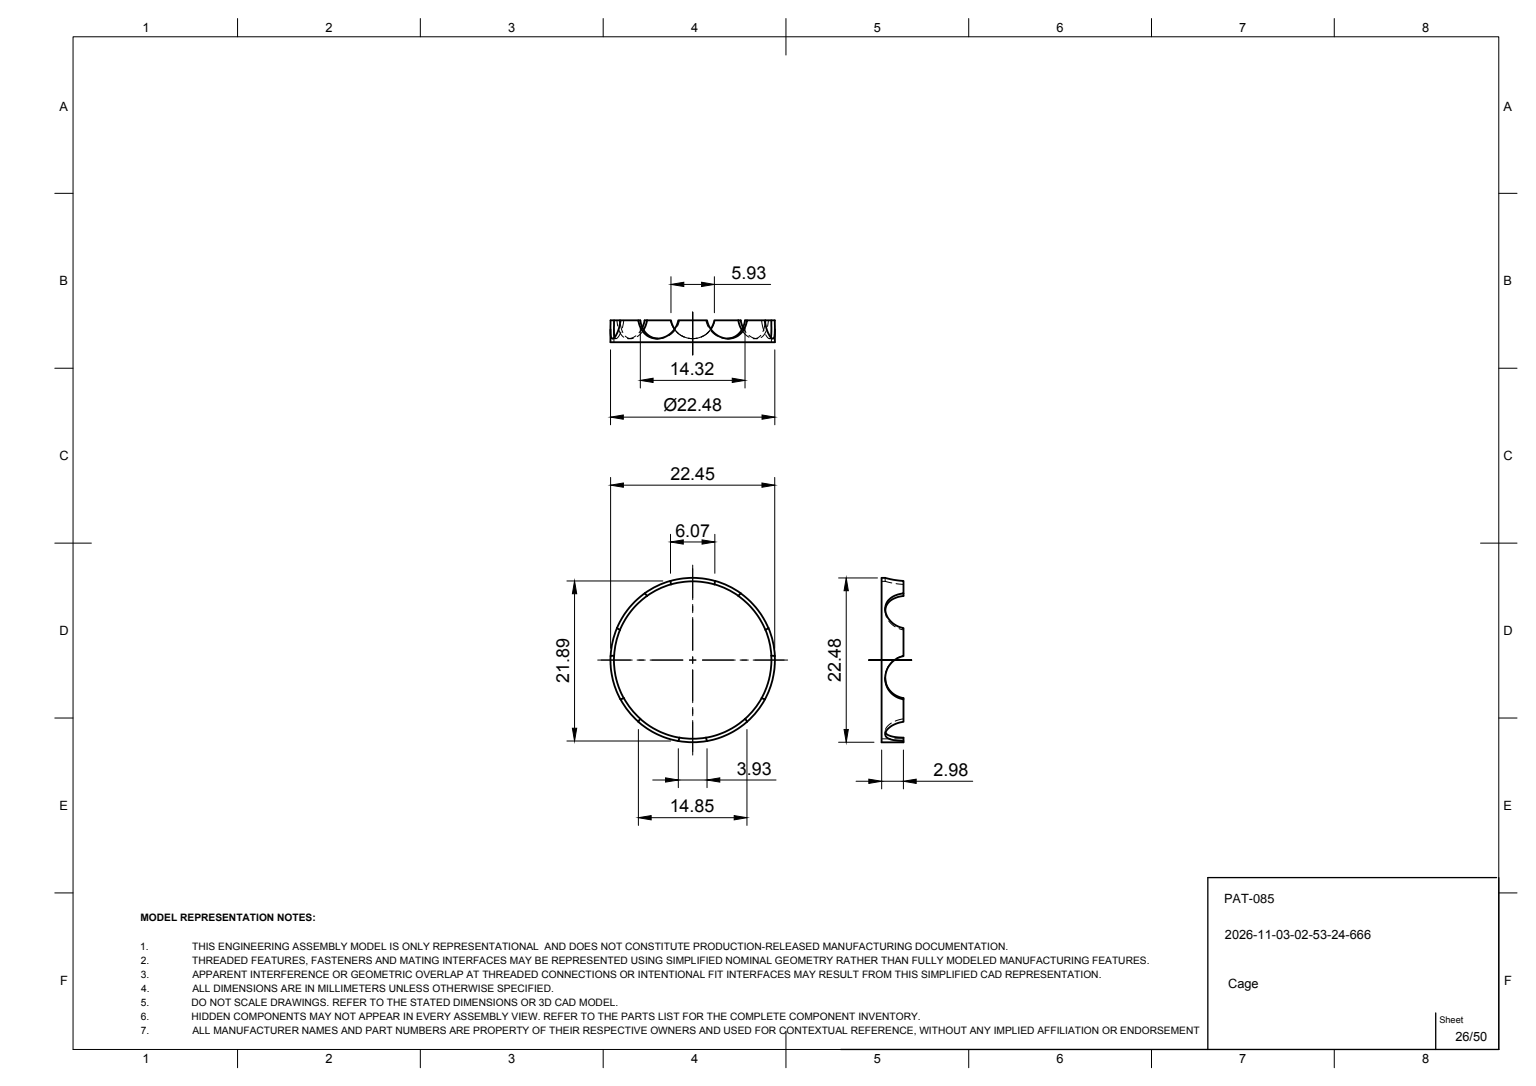
ISO-10303-21;
HEADER;
/* Generated by software containing ST-Developer
 * from STEP Tools, Inc. (www.steptools.com) 
 */

FILE_DESCRIPTION(
/* description */ ('Rack and pinion manual slide'),
/* implementation_level */ '2;1');

FILE_NAME(
/* name */ 'Cage.step',
/* time_stamp */ '2026-10-28T03:22:49-07:00',
/* author */ (''),
/* organization */ (''),
/* preprocessor_version */ 'ST-DEVELOPER v20.2',
/* originating_system */ 'Autodesk Translation Framework v15.17.0.0',
/* authorisation */ '');

FILE_SCHEMA (('AUTOMOTIVE_DESIGN { 1 0 10303 214 3 1 1 }'));
ENDSEC;

DATA;
#10=MECHANICAL_DESIGN_GEOMETRIC_PRESENTATION_REPRESENTATION('',(#760),#34851);
#575=B_SPLINE_CURVE_WITH_KNOTS('',3,(#20890,#20891,#20892,#20893,#20894,
#20895,#20896,#20897,#20898,#20899,#20900,#20901,#20902,#20903,#20904,#20905,
#20906,#20907,#20908,#20909,#20910,#20911),.UNSPECIFIED.,.F.,.F.,(4,2,2,
2,2,2,2,2,2,2,4),(0.0591825211272536,0.157966726598481,0.236950089897721,
0.315933453196962,0.391576304923761,0.46721915665056,0.54286200837736,0.618504860104159,
0.697488223403399,0.77647158670264,0.875255792173867),.UNSPECIFIED.);
#576=B_SPLINE_CURVE_WITH_KNOTS('',3,(#20915,#20916,#20917,#20918,#20919,
#20920,#20921,#20922,#20923,#20924,#20925,#20926,#20927,#20928,#20929,#20930,
#20931,#20932,#20933,#20934,#20935,#20936),.UNSPECIFIED.,.F.,.F.,(4,2,2,
2,2,2,2,2,2,2,4),(0.0581119756758434,0.106553146291161,0.213106292582322,
0.30849933801665,0.386091982889075,0.4636846277615,0.541277272633925,0.61886991750635,
0.714262962940678,0.820816109231839,0.869257279847157),.UNSPECIFIED.);
#577=B_SPLINE_CURVE_WITH_KNOTS('',3,(#20942,#20943,#20944,#20945,#20946,
#20947,#20948,#20949,#20950,#20951,#20952,#20953,#20954,#20955,#20956,#20957,
#20958,#20959,#20960,#20961,#20962,#20963),.UNSPECIFIED.,.F.,.F.,(4,2,2,
2,2,2,2,2,2,2,4),(0.0581119756758434,0.106553146291161,0.213106292582322,
0.30849933801665,0.386091982889075,0.4636846277615,0.541277272633925,0.61886991750635,
0.714262962940679,0.820816109231839,0.869257279847157),.UNSPECIFIED.);
#578=B_SPLINE_CURVE_WITH_KNOTS('',3,(#20967,#20968,#20969,#20970,#20971,
#20972,#20973,#20974,#20975,#20976,#20977,#20978,#20979,#20980,#20981,#20982,
#20983,#20984,#20985,#20986,#20987,#20988),.UNSPECIFIED.,.F.,.F.,(4,2,2,
2,2,2,2,2,2,2,4),(0.0581119756758433,0.106553146291161,0.213106292582322,
0.308499338016649,0.386091982889075,0.4636846277615,0.541277272633925,0.61886991750635,
0.714262962940678,0.820816109231839,0.869257279847157),.UNSPECIFIED.);
#579=B_SPLINE_CURVE_WITH_KNOTS('',3,(#20997,#20998,#20999,#21000,#21001,
#21002,#21003,#21004,#21005,#21006,#21007,#21008,#21009,#21010,#21011,#21012,
#21013,#21014,#21015,#21016,#21017,#21018),.UNSPECIFIED.,.F.,.F.,(4,2,2,
2,2,2,2,2,2,2,4),(0.0581119756758433,0.106553146291161,0.213106292582322,
0.30849933801665,0.386091982889075,0.4636846277615,0.541277272633925,0.61886991750635,
0.714262962940678,0.820816109231839,0.869257279847157),.UNSPECIFIED.);
#580=B_SPLINE_CURVE_WITH_KNOTS('',3,(#21022,#21023,#21024,#21025,#21026,
#21027,#21028,#21029,#21030,#21031,#21032,#21033,#21034,#21035,#21036,#21037,
#21038,#21039,#21040,#21041,#21042,#21043),.UNSPECIFIED.,.F.,.F.,(4,2,2,
2,2,2,2,2,2,2,4),(0.0581119756758434,0.106553146291161,0.213106292582322,
0.30849933801665,0.386091982889075,0.4636846277615,0.541277272633925,0.61886991750635,
0.714262962940678,0.820816109231839,0.869257279847157),.UNSPECIFIED.);
#581=B_SPLINE_CURVE_WITH_KNOTS('',3,(#21047,#21048,#21049,#21050,#21051,
#21052,#21053,#21054,#21055,#21056,#21057,#21058,#21059,#21060,#21061,#21062,
#21063,#21064,#21065,#21066,#21067,#21068),.UNSPECIFIED.,.F.,.F.,(4,2,2,
2,2,2,2,2,2,2,4),(0.0581119756758434,0.106553146291161,0.213106292582322,
0.30849933801665,0.386091982889075,0.4636846277615,0.541277272633925,0.61886991750635,
0.714262962940678,0.820816109231839,0.869257279847157),.UNSPECIFIED.);
#582=B_SPLINE_CURVE_WITH_KNOTS('',3,(#21072,#21073,#21074,#21075,#21076,
#21077,#21078,#21079,#21080,#21081,#21082,#21083,#21084,#21085,#21086,#21087,
#21088,#21089,#21090,#21091,#21092,#21093),.UNSPECIFIED.,.F.,.F.,(4,2,2,
2,2,2,2,2,2,2,4),(0.0581119756758433,0.106553146291161,0.213106292582322,
0.30849933801665,0.386091982889075,0.4636846277615,0.541277272633925,0.61886991750635,
0.714262962940678,0.820816109231839,0.869257279847157),.UNSPECIFIED.);
#583=B_SPLINE_CURVE_WITH_KNOTS('',3,(#21101,#21102,#21103,#21104,#21105,
#21106,#21107,#21108,#21109,#21110,#21111,#21112,#21113,#21114,#21115,#21116,
#21117,#21118,#21119,#21120,#21121,#21122),.UNSPECIFIED.,.F.,.F.,(4,2,2,
2,2,2,2,2,2,2,4),(0.0591825211272536,0.157966726598481,0.236950089897721,
0.315933453196962,0.391576304923761,0.467219156650561,0.54286200837736,
0.618504860104159,0.697488223403399,0.77647158670264,0.875255792173867),
 .UNSPECIFIED.);
#584=B_SPLINE_CURVE_WITH_KNOTS('',3,(#21130,#21131,#21132,#21133,#21134,
#21135,#21136,#21137,#21138,#21139,#21140,#21141,#21142,#21143,#21144,#21145,
#21146,#21147,#21148,#21149,#21150,#21151),.UNSPECIFIED.,.F.,.F.,(4,2,2,
2,2,2,2,2,2,2,4),(0.0591825211272536,0.157966726598481,0.236950089897722,
0.315933453196962,0.391576304923761,0.467219156650561,0.54286200837736,
0.618504860104159,0.697488223403399,0.77647158670264,0.875255792173867),
 .UNSPECIFIED.);
#585=B_SPLINE_CURVE_WITH_KNOTS('',3,(#21161,#21162,#21163,#21164,#21165,
#21166,#21167,#21168,#21169,#21170,#21171,#21172,#21173,#21174,#21175,#21176,
#21177,#21178,#21179,#21180,#21181,#21182),.UNSPECIFIED.,.F.,.F.,(4,2,2,
2,2,2,2,2,2,2,4),(0.0591825211272536,0.157966726598481,0.236950089897721,
0.315933453196962,0.391576304923761,0.46721915665056,0.54286200837736,0.618504860104159,
0.697488223403399,0.77647158670264,0.875255792173867),.UNSPECIFIED.);
#586=B_SPLINE_CURVE_WITH_KNOTS('',3,(#21190,#21191,#21192,#21193,#21194,
#21195,#21196,#21197,#21198,#21199,#21200,#21201,#21202,#21203,#21204,#21205,
#21206,#21207,#21208,#21209,#21210,#21211),.UNSPECIFIED.,.F.,.F.,(4,2,2,
2,2,2,2,2,2,2,4),(0.0591825211272536,0.157966726598481,0.236950089897721,
0.315933453196962,0.391576304923761,0.46721915665056,0.542862008377359,
0.618504860104159,0.697488223403399,0.776471586702639,0.875255792173867),
 .UNSPECIFIED.);
#587=B_SPLINE_CURVE_WITH_KNOTS('',3,(#21219,#21220,#21221,#21222,#21223,
#21224,#21225,#21226,#21227,#21228,#21229,#21230,#21231,#21232,#21233,#21234,
#21235,#21236,#21237,#21238,#21239,#21240),.UNSPECIFIED.,.F.,.F.,(4,2,2,
2,2,2,2,2,2,2,4),(0.0591825211272536,0.157966726598481,0.236950089897721,
0.315933453196962,0.391576304923761,0.46721915665056,0.54286200837736,0.618504860104159,
0.697488223403399,0.77647158670264,0.875255792173867),.UNSPECIFIED.);
#588=B_SPLINE_CURVE_WITH_KNOTS('',3,(#21249,#21250,#21251,#21252,#21253,
#21254,#21255,#21256,#21257,#21258,#21259,#21260,#21261,#21262,#21263,#21264,
#21265,#21266,#21267,#21268,#21269,#21270),.UNSPECIFIED.,.F.,.F.,(4,2,2,
2,2,2,2,2,2,2,4),(0.0591825211272536,0.157966726598481,0.236950089897721,
0.315933453196962,0.391576304923761,0.46721915665056,0.542862008377359,
0.618504860104159,0.697488223403399,0.776471586702639,0.875255792173867),
 .UNSPECIFIED.);
#596=SPHERICAL_SURFACE('',#14835,0.309556);
#597=SPHERICAL_SURFACE('',#14851,0.309556);
#598=SPHERICAL_SURFACE('',#14856,0.309556);
#599=SPHERICAL_SURFACE('',#14862,0.309556);
#600=SPHERICAL_SURFACE('',#14867,0.309556);
#601=SPHERICAL_SURFACE('',#14872,0.309556);
#602=SPHERICAL_SURFACE('',#14880,0.309556);
#662=SHAPE_REPRESENTATION_RELATIONSHIP('SRR','None',#35098,#708);
#708=ADVANCED_BREP_SHAPE_REPRESENTATION('',(#812),#34823);
#760=STYLED_ITEM('',(#35411),#812);
#812=MANIFOLD_SOLID_BREP('Continuous crown cage',#13781);
#979=FACE_BOUND('',#2722,.T.);
#1222=PLANE('',#14848);
#1223=PLANE('',#14853);
#1224=PLANE('',#14858);
#1225=PLANE('',#14864);
#1226=PLANE('',#14869);
#1227=PLANE('',#14878);
#1228=PLANE('',#14882);
#1229=PLANE('',#14883);
#1821=FACE_OUTER_BOUND('',#2706,.T.);
#1822=FACE_OUTER_BOUND('',#2707,.T.);
#1823=FACE_OUTER_BOUND('',#2708,.T.);
#1824=FACE_OUTER_BOUND('',#2709,.T.);
#1825=FACE_OUTER_BOUND('',#2710,.T.);
#1826=FACE_OUTER_BOUND('',#2711,.T.);
#1827=FACE_OUTER_BOUND('',#2712,.T.);
#1828=FACE_OUTER_BOUND('',#2713,.T.);
#1829=FACE_OUTER_BOUND('',#2714,.T.);
#1830=FACE_OUTER_BOUND('',#2715,.T.);
#1831=FACE_OUTER_BOUND('',#2716,.T.);
#1832=FACE_OUTER_BOUND('',#2717,.T.);
#1833=FACE_OUTER_BOUND('',#2718,.T.);
#1834=FACE_OUTER_BOUND('',#2719,.T.);
#1835=FACE_OUTER_BOUND('',#2720,.T.);
#1836=FACE_OUTER_BOUND('',#2721,.T.);
#1837=FACE_OUTER_BOUND('',#2723,.T.);
#2706=EDGE_LOOP('',(#10568,#10569,#10570,#10571));
#2707=EDGE_LOOP('',(#10572,#10573,#10574,#10575,#10576,#10577,#10578,#10579,
#10580,#10581,#10582,#10583,#10584,#10585,#10586,#10587,#10588,#10589));
#2708=EDGE_LOOP('',(#10590,#10591,#10592,#10593));
#2709=EDGE_LOOP('',(#10594,#10595,#10596,#10597));
#2710=EDGE_LOOP('',(#10598,#10599,#10600,#10601));
#2711=EDGE_LOOP('',(#10602,#10603,#10604,#10605));
#2712=EDGE_LOOP('',(#10606,#10607,#10608,#10609,#10610,#10611));
#2713=EDGE_LOOP('',(#10612,#10613,#10614,#10615));
#2714=EDGE_LOOP('',(#10616,#10617,#10618,#10619));
#2715=EDGE_LOOP('',(#10620,#10621,#10622,#10623));
#2716=EDGE_LOOP('',(#10624,#10625,#10626,#10627));
#2717=EDGE_LOOP('',(#10628,#10629,#10630,#10631));
#2718=EDGE_LOOP('',(#10632,#10633,#10634,#10635,#10636,#10637,#10638,#10639,
#10640,#10641,#10642,#10643,#10644,#10645,#10646,#10647,#10648,#10649));
#2719=EDGE_LOOP('',(#10650,#10651,#10652,#10653));
#2720=EDGE_LOOP('',(#10654,#10655,#10656,#10657));
#2721=EDGE_LOOP('',(#10658));
#2722=EDGE_LOOP('',(#10659));
#2723=EDGE_LOOP('',(#10660,#10661,#10662,#10663));
#3685=LINE('',#20992,#4976);
#3686=LINE('',#21245,#4977);
#4976=VECTOR('',#17111,1.123812);
#4977=VECTOR('',#17180,1.076188);
#6010=CIRCLE('',#14836,0.303778037777585);
#6011=CIRCLE('',#14837,0.303778037777585);
#6012=CIRCLE('',#14839,1.123812);
#6013=CIRCLE('',#14840,1.123812);
#6014=CIRCLE('',#14841,1.123812);
#6015=CIRCLE('',#14842,1.123812);
#6016=CIRCLE('',#14843,1.123812);
#6017=CIRCLE('',#14844,1.123812);
#6018=CIRCLE('',#14845,1.123812);
#6019=CIRCLE('',#14846,1.123812);
#6020=CIRCLE('',#14847,1.123812);
#6021=CIRCLE('',#14849,1.076188);
#6022=CIRCLE('',#14850,0.303778037777585);
#6023=CIRCLE('',#14852,0.303778037777585);
#6024=CIRCLE('',#14854,1.076188);
#6025=CIRCLE('',#14855,0.303778037777585);
#6026=CIRCLE('',#14857,0.303778037777585);
#6027=CIRCLE('',#14859,1.076188);
#6028=CIRCLE('',#14860,1.076188);
#6029=CIRCLE('',#14861,0.303778037777585);
#6030=CIRCLE('',#14863,0.303778037777585);
#6031=CIRCLE('',#14865,1.076188);
#6032=CIRCLE('',#14866,0.303778037777585);
#6033=CIRCLE('',#14868,0.303778037777585);
#6034=CIRCLE('',#14870,1.076188);
#6035=CIRCLE('',#14871,0.303778037777585);
#6036=CIRCLE('',#14873,0.303778037777585);
#6037=CIRCLE('',#14875,1.076188);
#6038=CIRCLE('',#14876,1.076188);
#6039=CIRCLE('',#14877,1.076188);
#6040=CIRCLE('',#14879,0.303778037777585);
#6041=CIRCLE('',#14881,0.303778037777585);
#6675=VERTEX_POINT('',#20888);
#6676=VERTEX_POINT('',#20889);
#6677=VERTEX_POINT('',#20912);
#6678=VERTEX_POINT('',#20914);
#6679=VERTEX_POINT('',#20939);
#6680=VERTEX_POINT('',#20941);
#6681=VERTEX_POINT('',#20964);
#6682=VERTEX_POINT('',#20966);
#6683=VERTEX_POINT('',#20989);
#6684=VERTEX_POINT('',#20991);
#6685=VERTEX_POINT('',#20994);
#6686=VERTEX_POINT('',#20996);
#6687=VERTEX_POINT('',#21019);
#6688=VERTEX_POINT('',#21021);
#6689=VERTEX_POINT('',#21044);
#6690=VERTEX_POINT('',#21046);
#6691=VERTEX_POINT('',#21069);
#6692=VERTEX_POINT('',#21071);
#6693=VERTEX_POINT('',#21096);
#6694=VERTEX_POINT('',#21100);
#6695=VERTEX_POINT('',#21125);
#6696=VERTEX_POINT('',#21129);
#6697=VERTEX_POINT('',#21154);
#6698=VERTEX_POINT('',#21156);
#6699=VERTEX_POINT('',#21160);
#6700=VERTEX_POINT('',#21185);
#6701=VERTEX_POINT('',#21189);
#6702=VERTEX_POINT('',#21214);
#6703=VERTEX_POINT('',#21218);
#6704=VERTEX_POINT('',#21243);
#6705=VERTEX_POINT('',#21246);
#6706=VERTEX_POINT('',#21248);
#8096=EDGE_CURVE('',#6675,#6676,#575,.T.);
#8097=EDGE_CURVE('',#6677,#6675,#6010,.T.);
#8098=EDGE_CURVE('',#6678,#6677,#576,.T.);
#8099=EDGE_CURVE('',#6676,#6678,#6011,.T.);
#8100=EDGE_CURVE('',#6679,#6677,#6012,.T.);
#8101=EDGE_CURVE('',#6679,#6680,#577,.T.);
#8102=EDGE_CURVE('',#6681,#6680,#6013,.T.);
#8103=EDGE_CURVE('',#6681,#6682,#578,.T.);
#8104=EDGE_CURVE('',#6683,#6682,#6014,.T.);
#8105=EDGE_CURVE('',#6683,#6684,#3685,.T.);
#8106=EDGE_CURVE('',#6684,#6684,#6015,.T.);
#8107=EDGE_CURVE('',#6685,#6683,#6016,.T.);
#8108=EDGE_CURVE('',#6685,#6686,#579,.T.);
#8109=EDGE_CURVE('',#6687,#6686,#6017,.T.);
#8110=EDGE_CURVE('',#6687,#6688,#580,.T.);
#8111=EDGE_CURVE('',#6689,#6688,#6018,.T.);
#8112=EDGE_CURVE('',#6689,#6690,#581,.T.);
#8113=EDGE_CURVE('',#6691,#6690,#6019,.T.);
#8114=EDGE_CURVE('',#6691,#6692,#582,.T.);
#8115=EDGE_CURVE('',#6678,#6692,#6020,.T.);
#8116=EDGE_CURVE('',#6675,#6693,#6021,.T.);
#8117=EDGE_CURVE('',#6693,#6679,#6022,.T.);
#8118=EDGE_CURVE('',#6694,#6693,#583,.T.);
#8119=EDGE_CURVE('',#6680,#6694,#6023,.T.);
#8120=EDGE_CURVE('',#6694,#6695,#6024,.T.);
#8121=EDGE_CURVE('',#6695,#6681,#6025,.T.);
#8122=EDGE_CURVE('',#6696,#6695,#584,.T.);
#8123=EDGE_CURVE('',#6682,#6696,#6026,.T.);
#8124=EDGE_CURVE('',#6696,#6697,#6027,.T.);
#8125=EDGE_CURVE('',#6697,#6698,#6028,.T.);
#8126=EDGE_CURVE('',#6698,#6685,#6029,.T.);
#8127=EDGE_CURVE('',#6699,#6698,#585,.T.);
#8128=EDGE_CURVE('',#6686,#6699,#6030,.T.);
#8129=EDGE_CURVE('',#6699,#6700,#6031,.T.);
#8130=EDGE_CURVE('',#6700,#6687,#6032,.T.);
#8131=EDGE_CURVE('',#6701,#6700,#586,.T.);
#8132=EDGE_CURVE('',#6688,#6701,#6033,.T.);
#8133=EDGE_CURVE('',#6701,#6702,#6034,.T.);
#8134=EDGE_CURVE('',#6702,#6689,#6035,.T.);
#8135=EDGE_CURVE('',#6703,#6702,#587,.T.);
#8136=EDGE_CURVE('',#6690,#6703,#6036,.T.);
#8137=EDGE_CURVE('',#6704,#6704,#6037,.T.);
#8138=EDGE_CURVE('',#6704,#6697,#3686,.T.);
#8139=EDGE_CURVE('',#6705,#6676,#6038,.T.);
#8140=EDGE_CURVE('',#6705,#6706,#588,.T.);
#8141=EDGE_CURVE('',#6703,#6706,#6039,.T.);
#8142=EDGE_CURVE('',#6692,#6705,#6040,.T.);
#8143=EDGE_CURVE('',#6706,#6691,#6041,.T.);
#10568=ORIENTED_EDGE('',*,*,#8096,.F.);
#10569=ORIENTED_EDGE('',*,*,#8097,.F.);
#10570=ORIENTED_EDGE('',*,*,#8098,.F.);
#10571=ORIENTED_EDGE('',*,*,#8099,.F.);
#10572=ORIENTED_EDGE('',*,*,#8098,.T.);
#10573=ORIENTED_EDGE('',*,*,#8100,.F.);
#10574=ORIENTED_EDGE('',*,*,#8101,.T.);
#10575=ORIENTED_EDGE('',*,*,#8102,.F.);
#10576=ORIENTED_EDGE('',*,*,#8103,.T.);
#10577=ORIENTED_EDGE('',*,*,#8104,.F.);
#10578=ORIENTED_EDGE('',*,*,#8105,.T.);
#10579=ORIENTED_EDGE('',*,*,#8106,.F.);
#10580=ORIENTED_EDGE('',*,*,#8105,.F.);
#10581=ORIENTED_EDGE('',*,*,#8107,.F.);
#10582=ORIENTED_EDGE('',*,*,#8108,.T.);
#10583=ORIENTED_EDGE('',*,*,#8109,.F.);
#10584=ORIENTED_EDGE('',*,*,#8110,.T.);
#10585=ORIENTED_EDGE('',*,*,#8111,.F.);
#10586=ORIENTED_EDGE('',*,*,#8112,.T.);
#10587=ORIENTED_EDGE('',*,*,#8113,.F.);
#10588=ORIENTED_EDGE('',*,*,#8114,.T.);
#10589=ORIENTED_EDGE('',*,*,#8115,.F.);
#10590=ORIENTED_EDGE('',*,*,#8097,.T.);
#10591=ORIENTED_EDGE('',*,*,#8116,.T.);
#10592=ORIENTED_EDGE('',*,*,#8117,.T.);
#10593=ORIENTED_EDGE('',*,*,#8100,.T.);
#10594=ORIENTED_EDGE('',*,*,#8118,.F.);
#10595=ORIENTED_EDGE('',*,*,#8119,.F.);
#10596=ORIENTED_EDGE('',*,*,#8101,.F.);
#10597=ORIENTED_EDGE('',*,*,#8117,.F.);
#10598=ORIENTED_EDGE('',*,*,#8119,.T.);
#10599=ORIENTED_EDGE('',*,*,#8120,.T.);
#10600=ORIENTED_EDGE('',*,*,#8121,.T.);
#10601=ORIENTED_EDGE('',*,*,#8102,.T.);
#10602=ORIENTED_EDGE('',*,*,#8122,.F.);
#10603=ORIENTED_EDGE('',*,*,#8123,.F.);
#10604=ORIENTED_EDGE('',*,*,#8103,.F.);
#10605=ORIENTED_EDGE('',*,*,#8121,.F.);
#10606=ORIENTED_EDGE('',*,*,#8123,.T.);
#10607=ORIENTED_EDGE('',*,*,#8124,.T.);
#10608=ORIENTED_EDGE('',*,*,#8125,.T.);
#10609=ORIENTED_EDGE('',*,*,#8126,.T.);
#10610=ORIENTED_EDGE('',*,*,#8107,.T.);
#10611=ORIENTED_EDGE('',*,*,#8104,.T.);
#10612=ORIENTED_EDGE('',*,*,#8127,.F.);
#10613=ORIENTED_EDGE('',*,*,#8128,.F.);
#10614=ORIENTED_EDGE('',*,*,#8108,.F.);
#10615=ORIENTED_EDGE('',*,*,#8126,.F.);
#10616=ORIENTED_EDGE('',*,*,#8128,.T.);
#10617=ORIENTED_EDGE('',*,*,#8129,.T.);
#10618=ORIENTED_EDGE('',*,*,#8130,.T.);
#10619=ORIENTED_EDGE('',*,*,#8109,.T.);
#10620=ORIENTED_EDGE('',*,*,#8131,.F.);
#10621=ORIENTED_EDGE('',*,*,#8132,.F.);
#10622=ORIENTED_EDGE('',*,*,#8110,.F.);
#10623=ORIENTED_EDGE('',*,*,#8130,.F.);
#10624=ORIENTED_EDGE('',*,*,#8132,.T.);
#10625=ORIENTED_EDGE('',*,*,#8133,.T.);
#10626=ORIENTED_EDGE('',*,*,#8134,.T.);
#10627=ORIENTED_EDGE('',*,*,#8111,.T.);
#10628=ORIENTED_EDGE('',*,*,#8112,.F.);
#10629=ORIENTED_EDGE('',*,*,#8134,.F.);
#10630=ORIENTED_EDGE('',*,*,#8135,.F.);
#10631=ORIENTED_EDGE('',*,*,#8136,.F.);
#10632=ORIENTED_EDGE('',*,*,#8137,.F.);
#10633=ORIENTED_EDGE('',*,*,#8138,.T.);
#10634=ORIENTED_EDGE('',*,*,#8124,.F.);
#10635=ORIENTED_EDGE('',*,*,#8122,.T.);
#10636=ORIENTED_EDGE('',*,*,#8120,.F.);
#10637=ORIENTED_EDGE('',*,*,#8118,.T.);
#10638=ORIENTED_EDGE('',*,*,#8116,.F.);
#10639=ORIENTED_EDGE('',*,*,#8096,.T.);
#10640=ORIENTED_EDGE('',*,*,#8139,.F.);
#10641=ORIENTED_EDGE('',*,*,#8140,.T.);
#10642=ORIENTED_EDGE('',*,*,#8141,.F.);
#10643=ORIENTED_EDGE('',*,*,#8135,.T.);
#10644=ORIENTED_EDGE('',*,*,#8133,.F.);
#10645=ORIENTED_EDGE('',*,*,#8131,.T.);
#10646=ORIENTED_EDGE('',*,*,#8129,.F.);
#10647=ORIENTED_EDGE('',*,*,#8127,.T.);
#10648=ORIENTED_EDGE('',*,*,#8125,.F.);
#10649=ORIENTED_EDGE('',*,*,#8138,.F.);
#10650=ORIENTED_EDGE('',*,*,#8099,.T.);
#10651=ORIENTED_EDGE('',*,*,#8115,.T.);
#10652=ORIENTED_EDGE('',*,*,#8142,.T.);
#10653=ORIENTED_EDGE('',*,*,#8139,.T.);
#10654=ORIENTED_EDGE('',*,*,#8114,.F.);
#10655=ORIENTED_EDGE('',*,*,#8143,.F.);
#10656=ORIENTED_EDGE('',*,*,#8140,.F.);
#10657=ORIENTED_EDGE('',*,*,#8142,.F.);
#10658=ORIENTED_EDGE('',*,*,#8106,.T.);
#10659=ORIENTED_EDGE('',*,*,#8137,.T.);
#10660=ORIENTED_EDGE('',*,*,#8136,.T.);
#10661=ORIENTED_EDGE('',*,*,#8141,.T.);
#10662=ORIENTED_EDGE('',*,*,#8143,.T.);
#10663=ORIENTED_EDGE('',*,*,#8113,.T.);
#12934=CYLINDRICAL_SURFACE('',#14838,1.123812);
#12935=CYLINDRICAL_SURFACE('',#14874,1.076188);
#13299=ADVANCED_FACE('',(#1821),#596,.F.);
#13300=ADVANCED_FACE('',(#1822),#12934,.T.);
#13301=ADVANCED_FACE('',(#1823),#1222,.T.);
#13302=ADVANCED_FACE('',(#1824),#597,.F.);
#13303=ADVANCED_FACE('',(#1825),#1223,.T.);
#13304=ADVANCED_FACE('',(#1826),#598,.F.);
#13305=ADVANCED_FACE('',(#1827),#1224,.T.);
#13306=ADVANCED_FACE('',(#1828),#599,.F.);
#13307=ADVANCED_FACE('',(#1829),#1225,.T.);
#13308=ADVANCED_FACE('',(#1830),#600,.F.);
#13309=ADVANCED_FACE('',(#1831),#1226,.T.);
#13310=ADVANCED_FACE('',(#1832),#601,.F.);
#13311=ADVANCED_FACE('',(#1833),#12935,.F.);
#13312=ADVANCED_FACE('',(#1834),#1227,.T.);
#13313=ADVANCED_FACE('',(#1835),#602,.F.);
#13314=ADVANCED_FACE('',(#1836,#979),#1228,.T.);
#13315=ADVANCED_FACE('',(#1837),#1229,.T.);
#13781=CLOSED_SHELL('',(#13299,#13300,#13301,#13302,#13303,#13304,#13305,
#13306,#13307,#13308,#13309,#13310,#13311,#13312,#13313,#13314,#13315));
#14834=AXIS2_PLACEMENT_3D('',#20886,#17095,#17096);
#14835=AXIS2_PLACEMENT_3D('',#20887,#17097,#17098);
#14836=AXIS2_PLACEMENT_3D('',#20913,#17099,#17100);
#14837=AXIS2_PLACEMENT_3D('',#20937,#17101,#17102);
#14838=AXIS2_PLACEMENT_3D('',#20938,#17103,#17104);
#14839=AXIS2_PLACEMENT_3D('',#20940,#17105,#17106);
#14840=AXIS2_PLACEMENT_3D('',#20965,#17107,#17108);
#14841=AXIS2_PLACEMENT_3D('',#20990,#17109,#17110);
#14842=AXIS2_PLACEMENT_3D('',#20993,#17112,#17113);
#14843=AXIS2_PLACEMENT_3D('',#20995,#17114,#17115);
#14844=AXIS2_PLACEMENT_3D('',#21020,#17116,#17117);
#14845=AXIS2_PLACEMENT_3D('',#21045,#17118,#17119);
#14846=AXIS2_PLACEMENT_3D('',#21070,#17120,#17121);
#14847=AXIS2_PLACEMENT_3D('',#21094,#17122,#17123);
#14848=AXIS2_PLACEMENT_3D('',#21095,#17124,#17125);
#14849=AXIS2_PLACEMENT_3D('',#21097,#17126,#17127);
#14850=AXIS2_PLACEMENT_3D('',#21098,#17128,#17129);
#14851=AXIS2_PLACEMENT_3D('',#21099,#17130,#17131);
#14852=AXIS2_PLACEMENT_3D('',#21123,#17132,#17133);
#14853=AXIS2_PLACEMENT_3D('',#21124,#17134,#17135);
#14854=AXIS2_PLACEMENT_3D('',#21126,#17136,#17137);
#14855=AXIS2_PLACEMENT_3D('',#21127,#17138,#17139);
#14856=AXIS2_PLACEMENT_3D('',#21128,#17140,#17141);
#14857=AXIS2_PLACEMENT_3D('',#21152,#17142,#17143);
#14858=AXIS2_PLACEMENT_3D('',#21153,#17144,#17145);
#14859=AXIS2_PLACEMENT_3D('',#21155,#17146,#17147);
#14860=AXIS2_PLACEMENT_3D('',#21157,#17148,#17149);
#14861=AXIS2_PLACEMENT_3D('',#21158,#17150,#17151);
#14862=AXIS2_PLACEMENT_3D('',#21159,#17152,#17153);
#14863=AXIS2_PLACEMENT_3D('',#21183,#17154,#17155);
#14864=AXIS2_PLACEMENT_3D('',#21184,#17156,#17157);
#14865=AXIS2_PLACEMENT_3D('',#21186,#17158,#17159);
#14866=AXIS2_PLACEMENT_3D('',#21187,#17160,#17161);
#14867=AXIS2_PLACEMENT_3D('',#21188,#17162,#17163);
#14868=AXIS2_PLACEMENT_3D('',#21212,#17164,#17165);
#14869=AXIS2_PLACEMENT_3D('',#21213,#17166,#17167);
#14870=AXIS2_PLACEMENT_3D('',#21215,#17168,#17169);
#14871=AXIS2_PLACEMENT_3D('',#21216,#17170,#17171);
#14872=AXIS2_PLACEMENT_3D('',#21217,#17172,#17173);
#14873=AXIS2_PLACEMENT_3D('',#21241,#17174,#17175);
#14874=AXIS2_PLACEMENT_3D('',#21242,#17176,#17177);
#14875=AXIS2_PLACEMENT_3D('',#21244,#17178,#17179);
#14876=AXIS2_PLACEMENT_3D('',#21247,#17181,#17182);
#14877=AXIS2_PLACEMENT_3D('',#21271,#17183,#17184);
#14878=AXIS2_PLACEMENT_3D('',#21272,#17185,#17186);
#14879=AXIS2_PLACEMENT_3D('',#21273,#17187,#17188);
#14880=AXIS2_PLACEMENT_3D('',#21274,#17189,#17190);
#14881=AXIS2_PLACEMENT_3D('',#21275,#17191,#17192);
#14882=AXIS2_PLACEMENT_3D('',#21276,#17193,#17194);
#14883=AXIS2_PLACEMENT_3D('',#21277,#17195,#17196);
#17095=DIRECTION('axis',(0.,0.,1.));
#17096=DIRECTION('refdir',(1.,0.,0.));
#17097=DIRECTION('center_axis',(0.,0.,1.));
#17098=DIRECTION('ref_axis',(1.,0.,0.));
#17099=DIRECTION('center_axis',(0.,-1.,0.));
#17100=DIRECTION('ref_axis',(0.,0.,-1.));
#17101=DIRECTION('center_axis',(0.,-1.,0.));
#17102=DIRECTION('ref_axis',(0.,0.,-1.));
#17103=DIRECTION('center_axis',(0.,1.,0.));
#17104=DIRECTION('ref_axis',(1.,0.,0.));
#17105=DIRECTION('center_axis',(0.,1.,0.));
#17106=DIRECTION('ref_axis',(1.,0.,0.));
#17107=DIRECTION('center_axis',(0.,1.,0.));
#17108=DIRECTION('ref_axis',(1.,0.,0.));
#17109=DIRECTION('center_axis',(0.,1.,0.));
#17110=DIRECTION('ref_axis',(1.,0.,0.));
#17111=DIRECTION('',(0.,-1.,0.));
#17112=DIRECTION('center_axis',(0.,-1.,0.));
#17113=DIRECTION('ref_axis',(1.,0.,0.));
#17114=DIRECTION('center_axis',(0.,1.,0.));
#17115=DIRECTION('ref_axis',(1.,0.,0.));
#17116=DIRECTION('center_axis',(0.,1.,0.));
#17117=DIRECTION('ref_axis',(1.,0.,0.));
#17118=DIRECTION('center_axis',(0.,1.,0.));
#17119=DIRECTION('ref_axis',(1.,0.,0.));
#17120=DIRECTION('center_axis',(0.,1.,0.));
#17121=DIRECTION('ref_axis',(1.,0.,0.));
#17122=DIRECTION('center_axis',(0.,1.,0.));
#17123=DIRECTION('ref_axis',(1.,0.,0.));
#17124=DIRECTION('center_axis',(0.,1.,0.));
#17125=DIRECTION('ref_axis',(1.,0.,0.));
#17126=DIRECTION('center_axis',(0.,-1.,0.));
#17127=DIRECTION('ref_axis',(1.,0.,0.));
#17128=DIRECTION('center_axis',(0.,-1.,0.));
#17129=DIRECTION('ref_axis',(0.,0.,-1.));
#17130=DIRECTION('center_axis',(8.96625347776458E-17,0.,1.));
#17131=DIRECTION('ref_axis',(1.,0.,0.));
#17132=DIRECTION('center_axis',(0.,-1.,0.));
#17133=DIRECTION('ref_axis',(0.,0.,-1.));
#17134=DIRECTION('center_axis',(0.,1.,0.));
#17135=DIRECTION('ref_axis',(1.,0.,0.));
#17136=DIRECTION('center_axis',(0.,-1.,0.));
#17137=DIRECTION('ref_axis',(1.,0.,0.));
#17138=DIRECTION('center_axis',(0.,-1.,0.));
#17139=DIRECTION('ref_axis',(0.,0.,-1.));
#17140=DIRECTION('center_axis',(0.,0.,1.));
#17141=DIRECTION('ref_axis',(1.,0.,0.));
#17142=DIRECTION('center_axis',(0.,-1.,0.));
#17143=DIRECTION('ref_axis',(0.,0.,-1.));
#17144=DIRECTION('center_axis',(0.,1.,0.));
#17145=DIRECTION('ref_axis',(1.,0.,0.));
#17146=DIRECTION('center_axis',(0.,-1.,0.));
#17147=DIRECTION('ref_axis',(1.,0.,0.));
#17148=DIRECTION('center_axis',(0.,-1.,0.));
#17149=DIRECTION('ref_axis',(1.,0.,0.));
#17150=DIRECTION('center_axis',(0.,-1.,0.));
#17151=DIRECTION('ref_axis',(0.,0.,-1.));
#17152=DIRECTION('center_axis',(0.,0.,1.));
#17153=DIRECTION('ref_axis',(1.,0.,0.));
#17154=DIRECTION('center_axis',(0.,-1.,0.));
#17155=DIRECTION('ref_axis',(0.,0.,-1.));
#17156=DIRECTION('center_axis',(0.,1.,0.));
#17157=DIRECTION('ref_axis',(1.,0.,0.));
#17158=DIRECTION('center_axis',(0.,-1.,0.));
#17159=DIRECTION('ref_axis',(1.,0.,0.));
#17160=DIRECTION('center_axis',(0.,-1.,0.));
#17161=DIRECTION('ref_axis',(0.,0.,-1.));
#17162=DIRECTION('center_axis',(8.96625347776458E-17,0.,1.));
#17163=DIRECTION('ref_axis',(1.,0.,0.));
#17164=DIRECTION('center_axis',(0.,-1.,0.));
#17165=DIRECTION('ref_axis',(0.,0.,-1.));
#17166=DIRECTION('center_axis',(0.,1.,0.));
#17167=DIRECTION('ref_axis',(1.,0.,0.));
#17168=DIRECTION('center_axis',(0.,-1.,0.));
#17169=DIRECTION('ref_axis',(1.,0.,0.));
#17170=DIRECTION('center_axis',(0.,-1.,0.));
#17171=DIRECTION('ref_axis',(0.,0.,-1.));
#17172=DIRECTION('center_axis',(0.,0.,1.));
#17173=DIRECTION('ref_axis',(1.,0.,0.));
#17174=DIRECTION('center_axis',(0.,-1.,0.));
#17175=DIRECTION('ref_axis',(0.,0.,-1.));
#17176=DIRECTION('center_axis',(0.,1.,0.));
#17177=DIRECTION('ref_axis',(1.,0.,0.));
#17178=DIRECTION('center_axis',(0.,1.,0.));
#17179=DIRECTION('ref_axis',(1.,0.,0.));
#17180=DIRECTION('',(0.,1.,0.));
#17181=DIRECTION('center_axis',(0.,-1.,0.));
#17182=DIRECTION('ref_axis',(1.,0.,0.));
#17183=DIRECTION('center_axis',(0.,-1.,0.));
#17184=DIRECTION('ref_axis',(1.,0.,0.));
#17185=DIRECTION('center_axis',(0.,1.,0.));
#17186=DIRECTION('ref_axis',(1.,0.,0.));
#17187=DIRECTION('center_axis',(0.,-1.,0.));
#17188=DIRECTION('ref_axis',(0.,0.,-1.));
#17189=DIRECTION('center_axis',(0.,0.,1.));
#17190=DIRECTION('ref_axis',(1.,0.,0.));
#17191=DIRECTION('center_axis',(0.,-1.,0.));
#17192=DIRECTION('ref_axis',(0.,0.,-1.));
#17193=DIRECTION('center_axis',(0.,-1.,0.));
#17194=DIRECTION('ref_axis',(-1.,0.,0.));
#17195=DIRECTION('center_axis',(0.,1.,0.));
#17196=DIRECTION('ref_axis',(1.,0.,0.));
#20886=CARTESIAN_POINT('',(0.,0.,0.));
#20887=CARTESIAN_POINT('Origin',(0.685838782044607,0.,0.860014630714833));
#20888=CARTESIAN_POINT('',(0.413083465285518,-0.05953,0.993751811093549));
#20889=CARTESIAN_POINT('',(0.876916659919095,-0.05953,0.623857181492959));
#20890=CARTESIAN_POINT('Ctrl Pts',(0.413083465285518,-0.05953,0.993751811093549));
#20891=CARTESIAN_POINT('Ctrl Pts',(0.419070565453383,-0.0925528133349865,
0.991263089003441));
#20892=CARTESIAN_POINT('Ctrl Pts',(0.430199341854858,-0.124911173756694,
0.986608710139579));
#20893=CARTESIAN_POINT('Ctrl Pts',(0.457978755888596,-0.177924977804098,
0.973971221090534));
#20894=CARTESIAN_POINT('Ctrl Pts',(0.473077587363685,-0.199697230012983,
0.966820759530997));
#20895=CARTESIAN_POINT('Ctrl Pts',(0.507057380724533,-0.237895043532788,
0.949440676105255));
#20896=CARTESIAN_POINT('Ctrl Pts',(0.525933334162555,-0.254319232363049,
0.939198248544428));
#20897=CARTESIAN_POINT('Ctrl Pts',(0.564362943424238,-0.28018331644634,
0.916597376014514));
#20898=CARTESIAN_POINT('Ctrl Pts',(0.585840553788742,-0.29104845371857,
0.903141581680914));
#20899=CARTESIAN_POINT('Ctrl Pts',(0.629305439856167,-0.30527573347708,
0.873412008702649));
#20900=CARTESIAN_POINT('Ctrl Pts',(0.651278921914856,-0.308638795020976,
0.857118508332695));
#20901=CARTESIAN_POINT('Ctrl Pts',(0.690705563850638,-0.308638795020976,
0.825676810575914));
#20902=CARTESIAN_POINT('Ctrl Pts',(0.711480111898423,-0.30527573347708,
0.807879894508811));
#20903=CARTESIAN_POINT('Ctrl Pts',(0.750136149454208,-0.29104845371857,
0.772120216227122));
#20904=CARTESIAN_POINT('Ctrl Pts',(0.768033796848072,-0.28018331644634,
0.754175290318038));
#20905=CARTESIAN_POINT('Ctrl Pts',(0.798619410861634,-0.254319232363049,
0.721738358858166));
#20906=CARTESIAN_POINT('Ctrl Pts',(0.812805334167529,-0.237895043532788,
0.705614819529209));
#20907=CARTESIAN_POINT('Ctrl Pts',(0.837310877969633,-0.199697230012983,
0.676354402927683));
#20908=CARTESIAN_POINT('Ctrl Pts',(0.847641868610495,-0.177924977804098,
0.663225258065736));
#20909=CARTESIAN_POINT('Ctrl Pts',(0.866144010579847,-0.124911173756694,
0.638954437806245));
#20910=CARTESIAN_POINT('Ctrl Pts',(0.873158080166742,-0.0925528133349865,
0.62914037979579));
#20911=CARTESIAN_POINT('Ctrl Pts',(0.876916659919095,-0.05953,0.623857181492959));
#20912=CARTESIAN_POINT('',(0.437601487681057,-0.05953,1.03511272300331));
#20913=CARTESIAN_POINT('Origin',(0.685838782044607,-0.05953,0.860014630714833));
#20914=CARTESIAN_POINT('',(0.911784794170997,-0.05953,0.656964154625313));
#20915=CARTESIAN_POINT('Ctrl Pts',(0.911784794170998,-0.0595300000000001,
0.656964154625312));
#20916=CARTESIAN_POINT('Ctrl Pts',(0.909827729890942,-0.0762225747374255,
0.659680317203144));
#20917=CARTESIAN_POINT('Ctrl Pts',(0.907004864562642,-0.0928409665394228,
0.663576540841106));
#20918=CARTESIAN_POINT('Ctrl Pts',(0.895234408667242,-0.144299303100741,
0.679480524217551));
#20919=CARTESIAN_POINT('Ctrl Pts',(0.882797231409153,-0.177024326825049,
0.695831250979106));
#20920=CARTESIAN_POINT('Ctrl Pts',(0.854332839576145,-0.227269801620064,
0.73042219438957));
#20921=CARTESIAN_POINT('Ctrl Pts',(0.834863020612702,-0.251265615809407,
0.752807465209441));
#20922=CARTESIAN_POINT('Ctrl Pts',(0.800439809856111,-0.279889827963178,
0.789147407129766));
#20923=CARTESIAN_POINT('Ctrl Pts',(0.781998747691871,-0.290879136862659,
0.80756613568454));
#20924=CARTESIAN_POINT('Ctrl Pts',(0.742239891936898,-0.305251990234487,
0.844254137480382));
#20925=CARTESIAN_POINT('Ctrl Pts',(0.720906778729541,-0.308638795020976,
0.862505527716294));
#20926=CARTESIAN_POINT('Ctrl Pts',(0.680463863683392,-0.308638795020976,
0.894757676234429));
#20927=CARTESIAN_POINT('Ctrl Pts',(0.657923009631182,-0.305251990234488,
0.91149460735272));
#20928=CARTESIAN_POINT('Ctrl Pts',(0.613307674922609,-0.290879136862659,
0.942092777160053));
#20929=CARTESIAN_POINT('Ctrl Pts',(0.591247219971725,-0.279889827963178,
0.955972930713954));
#20930=CARTESIAN_POINT('Ctrl Pts',(0.548158511259202,-0.251265615809407,
0.981446681891443));
#20931=CARTESIAN_POINT('Ctrl Pts',(0.522002043615455,-0.227269801620063,
0.995447160474328));
#20932=CARTESIAN_POINT('Ctrl Pts',(0.481944444320713,-0.177024326825049,
1.01550068154148));
#20933=CARTESIAN_POINT('Ctrl Pts',(0.463236132117164,-0.14429930310074,
1.0239876538093));
#20934=CARTESIAN_POINT('Ctrl Pts',(0.445111721969657,-0.0928409665394226,
1.03192403056628));
#20935=CARTESIAN_POINT('Ctrl Pts',(0.440685038163619,-0.0762225747374254,
1.03380912944435));
#20936=CARTESIAN_POINT('Ctrl Pts',(0.437601487681056,-0.05953,1.03511272300331));
#20937=CARTESIAN_POINT('Origin',(0.685838782044607,-0.05953,0.860014630714833));
#20938=CARTESIAN_POINT('Origin',(0.,-0.208355,0.));
#20939=CARTESIAN_POINT('',(0.0548532617164168,-0.05953,1.12247250791415));
#20940=CARTESIAN_POINT('Origin',(0.,-0.05953,0.));
#20941=CARTESIAN_POINT('',(-0.536443649899848,-0.05953,0.987512846410683));
#20942=CARTESIAN_POINT('Ctrl Pts',(0.0548532617164173,-0.0595300000000001,
1.12247250791414));
#20943=CARTESIAN_POINT('Ctrl Pts',(0.05150947068137,-0.0762225747374254,
1.12263591311425));
#20944=CARTESIAN_POINT('Ctrl Pts',(0.0467032526342597,-0.0928409665394227,
1.12285816383385));
#20945=CARTESIAN_POINT('Ctrl Pts',(0.0269302585198975,-0.144299303100741,
1.12357162229597));
#20946=CARTESIAN_POINT('Ctrl Pts',(0.006392292392153,-0.177024326825049,
1.12404235695137));
#20947=CARTESIAN_POINT('Ctrl Pts',(-0.0383992541984087,-0.227269801620063,
1.12335509974011));
#20948=CARTESIAN_POINT('Ctrl Pts',(-0.0680399972366993,-0.251265615809407,
1.12208997038458));
#20949=CARTESIAN_POINT('Ctrl Pts',(-0.117914228755037,-0.279889827963178,
1.1178344036749));
#20950=CARTESIAN_POINT('Ctrl Pts',(-0.14381238480104,-0.290879136862659,
1.11490049012186));
#20951=CARTESIAN_POINT('Ctrl Pts',(-0.19728546073067,-0.305251990234488,
1.10669035995599));
#20952=CARTESIAN_POINT('Ctrl Pts',(-0.224855950742601,-0.308638795020976,
1.10139101611326));
#20953=CARTESIAN_POINT('Ctrl Pts',(-0.275287440920027,-0.308638795020976,
1.0898803575765));
#20954=CARTESIAN_POINT('Ctrl Pts',(-0.302426893214945,-0.305251990234488,
1.08269251410343));
#20955=CARTESIAN_POINT('Ctrl Pts',(-0.35416671187353,-0.290879136862659,
1.06688848765783));
#20956=CARTESIAN_POINT('Ctrl Pts',(-0.3787731215897,-0.279889827963178,
1.05829506364875));
#20957=CARTESIAN_POINT('Ctrl Pts',(-0.425554672694338,-0.251265615809407,
1.04048957871266));
#20958=CARTESIAN_POINT('Ctrl Pts',(-0.452808978448581,-0.227269801620063,
1.02876878445619));
#20959=CARTESIAN_POINT('Ctrl Pts',(-0.493462957200432,-0.177024326825049,
1.0099536580922));
#20960=CARTESIAN_POINT('Ctrl Pts',(-0.511762781179148,-0.14429930310074,
1.00061845128527));
#20961=CARTESIAN_POINT('Ctrl Pts',(-0.529268075276157,-0.0928409665394226,
0.991396466802468));
#20962=CARTESIAN_POINT('Ctrl Pts',(-0.533501897135713,-0.0762225747374254,
0.989110885965947));
#20963=CARTESIAN_POINT('Ctrl Pts',(-0.536443649899848,-0.0595300000000001,
0.987512846410683));
#20964=CARTESIAN_POINT('',(-0.843383895613249,-0.05953,0.742736168477219));
#20965=CARTESIAN_POINT('Origin',(0.,-0.05953,0.));
#20966=CARTESIAN_POINT('',(-1.10653577764992,-0.05953,0.196295654879792));
#20967=CARTESIAN_POINT('Ctrl Pts',(-0.843383895613249,-0.0595300000000001,
0.742736168477219));
#20968=CARTESIAN_POINT('Ctrl Pts',(-0.84559647055299,-0.0762225747374255,
0.740223768851062));
#20969=CARTESIAN_POINT('Ctrl Pts',(-0.848766861100456,-0.0928409665394227,
0.736604687327351));
#20970=CARTESIAN_POINT('Ctrl Pts',(-0.861652925570091,-0.144299303100741,
0.721590372101268));
#20971=CARTESIAN_POINT('Ctrl Pts',(-0.87482617317514,-0.177024326825049,
0.705826641853758));
#20972=CARTESIAN_POINT('Ctrl Pts',(-0.902215926359523,-0.227269801620063,
0.670378702718353));
#20973=CARTESIAN_POINT('Ctrl Pts',(-0.919707509403859,-0.251265615809407,
0.646415841396062));
#20974=CARTESIAN_POINT('Ctrl Pts',(-0.947476448101718,-0.279889827963178,
0.604769294586516));
#20975=CARTESIAN_POINT('Ctrl Pts',(-0.961329858300736,-0.290879136862659,
0.582692035672022));
#20976=CARTESIAN_POINT('Ctrl Pts',(-0.988250837578047,-0.305251990234488,
0.535766169015486));
#20977=CARTESIAN_POINT('Ctrl Pts',(-1.00129756308006,-0.308638795020976,
0.510906605094603));
#20978=CARTESIAN_POINT('Ctrl Pts',(-1.02374168767024,-0.308638795020976,
0.46430090015576));
#20979=CARTESIAN_POINT('Ctrl Pts',(-1.03504317708586,-0.305251990234488,
0.438600874831839));
#20980=CARTESIAN_POINT('Ctrl Pts',(-1.05494634094458,-0.290879136862659,
0.388295406390235));
#20981=CARTESIAN_POINT('Ctrl Pts',(-1.06356957703048,-0.279889827963178,
0.363699428370917));
#20982=CARTESIAN_POINT('Ctrl Pts',(-1.0788165083757,-0.251265615809407,
0.316022600643821));
#20983=CARTESIAN_POINT('Ctrl Pts',(-1.08664560412098,-0.227269801620063,
0.287406530683752));
#20984=CARTESIAN_POINT('Ctrl Pts',(-1.09728268713976,-0.177024326825049,
0.243890930799337));
#20985=CARTESIAN_POINT('Ctrl Pts',(-1.10139388218929,-0.144299303100741,
0.22376314604679));
#20986=CARTESIAN_POINT('Ctrl Pts',(-1.10509821673782,-0.0928409665394227,
0.204327142733961));
#20987=CARTESIAN_POINT('Ctrl Pts',(-1.10595102243643,-0.0762225747374254,
0.199591971170104));
#20988=CARTESIAN_POINT('Ctrl Pts',(-1.10653577764992,-0.0595300000000001,
0.196295654879792));
#20989=CARTESIAN_POINT('',(-1.123812,-0.05953,1.37627276864339E-16));
#20990=CARTESIAN_POINT('Origin',(0.,-0.05953,0.));
#20991=CARTESIAN_POINT('',(-1.123812,-0.35718,1.37627276864339E-16));
#20992=CARTESIAN_POINT('',(-1.123812,-0.208355,1.37627276864339E-16));
#20993=CARTESIAN_POINT('Origin',(0.,-0.35718,0.));
#20994=CARTESIAN_POINT('',(-1.10653577764992,-0.05953,-0.196295654879793));
#20995=CARTESIAN_POINT('Origin',(0.,-0.05953,0.));
#20996=CARTESIAN_POINT('',(-0.843383895613249,-0.05953,-0.742736168477219));
#20997=CARTESIAN_POINT('Ctrl Pts',(-1.10653577764992,-0.0595300000000001,
-0.196295654879792));
#20998=CARTESIAN_POINT('Ctrl Pts',(-1.10595102243643,-0.0762225747374255,
-0.199591971170104));
#20999=CARTESIAN_POINT('Ctrl Pts',(-1.10509821673782,-0.0928409665394228,
-0.204327142733962));
#21000=CARTESIAN_POINT('Ctrl Pts',(-1.10139388218929,-0.144299303100741,
-0.22376314604679));
#21001=CARTESIAN_POINT('Ctrl Pts',(-1.09728268713976,-0.177024326825049,
-0.243890930799338));
#21002=CARTESIAN_POINT('Ctrl Pts',(-1.08664560412098,-0.227269801620063,
-0.287406530683753));
#21003=CARTESIAN_POINT('Ctrl Pts',(-1.0788165083757,-0.251265615809407,
-0.316022600643821));
#21004=CARTESIAN_POINT('Ctrl Pts',(-1.06356957703048,-0.279889827963178,
-0.363699428370918));
#21005=CARTESIAN_POINT('Ctrl Pts',(-1.05494634094458,-0.290879136862659,
-0.388295406390235));
#21006=CARTESIAN_POINT('Ctrl Pts',(-1.03504317708586,-0.305251990234488,
-0.438600874831839));
#21007=CARTESIAN_POINT('Ctrl Pts',(-1.02374168767024,-0.308638795020976,
-0.46430090015576));
#21008=CARTESIAN_POINT('Ctrl Pts',(-1.00129756308006,-0.308638795020976,
-0.510906605094603));
#21009=CARTESIAN_POINT('Ctrl Pts',(-0.988250837578047,-0.305251990234488,
-0.535766169015486));
#21010=CARTESIAN_POINT('Ctrl Pts',(-0.961329858300736,-0.290879136862659,
-0.582692035672022));
#21011=CARTESIAN_POINT('Ctrl Pts',(-0.947476448101718,-0.279889827963178,
-0.604769294586516));
#21012=CARTESIAN_POINT('Ctrl Pts',(-0.919707509403859,-0.251265615809407,
-0.646415841396062));
#21013=CARTESIAN_POINT('Ctrl Pts',(-0.902215926359523,-0.227269801620064,
-0.670378702718353));
#21014=CARTESIAN_POINT('Ctrl Pts',(-0.87482617317514,-0.177024326825049,
-0.705826641853758));
#21015=CARTESIAN_POINT('Ctrl Pts',(-0.861652925570091,-0.144299303100741,
-0.721590372101268));
#21016=CARTESIAN_POINT('Ctrl Pts',(-0.848766861100456,-0.0928409665394229,
-0.736604687327351));
#21017=CARTESIAN_POINT('Ctrl Pts',(-0.84559647055299,-0.0762225747374255,
-0.740223768851063));
#21018=CARTESIAN_POINT('Ctrl Pts',(-0.843383895613249,-0.0595300000000001,
-0.742736168477219));
#21019=CARTESIAN_POINT('',(-0.536443649899847,-0.05953,-0.987512846410683));
#21020=CARTESIAN_POINT('Origin',(0.,-0.05953,0.));
#21021=CARTESIAN_POINT('',(0.0548532617164172,-0.05953,-1.12247250791415));
#21022=CARTESIAN_POINT('Ctrl Pts',(-0.536443649899848,-0.0595300000000001,
-0.987512846410683));
#21023=CARTESIAN_POINT('Ctrl Pts',(-0.533501897135712,-0.0762225747374254,
-0.989110885965947));
#21024=CARTESIAN_POINT('Ctrl Pts',(-0.529268075276156,-0.0928409665394227,
-0.991396466802469));
#21025=CARTESIAN_POINT('Ctrl Pts',(-0.511762781179147,-0.144299303100741,
-1.00061845128527));
#21026=CARTESIAN_POINT('Ctrl Pts',(-0.493462957200432,-0.177024326825049,
-1.0099536580922));
#21027=CARTESIAN_POINT('Ctrl Pts',(-0.45280897844858,-0.227269801620063,
-1.02876878445619));
#21028=CARTESIAN_POINT('Ctrl Pts',(-0.425554672694337,-0.251265615809407,
-1.04048957871266));
#21029=CARTESIAN_POINT('Ctrl Pts',(-0.3787731215897,-0.279889827963178,
-1.05829506364875));
#21030=CARTESIAN_POINT('Ctrl Pts',(-0.354166711873529,-0.290879136862659,
-1.06688848765783));
#21031=CARTESIAN_POINT('Ctrl Pts',(-0.302426893214944,-0.305251990234488,
-1.08269251410343));
#21032=CARTESIAN_POINT('Ctrl Pts',(-0.275287440920027,-0.308638795020976,
-1.0898803575765));
#21033=CARTESIAN_POINT('Ctrl Pts',(-0.224855950742601,-0.308638795020976,
-1.10139101611326));
#21034=CARTESIAN_POINT('Ctrl Pts',(-0.19728546073067,-0.305251990234488,
-1.10669035995599));
#21035=CARTESIAN_POINT('Ctrl Pts',(-0.143812384801039,-0.290879136862659,
-1.11490049012186));
#21036=CARTESIAN_POINT('Ctrl Pts',(-0.117914228755037,-0.279889827963178,
-1.1178344036749));
#21037=CARTESIAN_POINT('Ctrl Pts',(-0.0680399972366989,-0.251265615809407,
-1.12208997038458));
#21038=CARTESIAN_POINT('Ctrl Pts',(-0.0383992541984084,-0.227269801620063,
-1.12335509974011));
#21039=CARTESIAN_POINT('Ctrl Pts',(0.00639229239215326,-0.177024326825049,
-1.12404235695137));
#21040=CARTESIAN_POINT('Ctrl Pts',(0.0269302585198977,-0.144299303100741,
-1.12357162229597));
#21041=CARTESIAN_POINT('Ctrl Pts',(0.04670325263426,-0.0928409665394228,
-1.12285816383385));
#21042=CARTESIAN_POINT('Ctrl Pts',(0.0515094706813703,-0.0762225747374255,
-1.12263591311425));
#21043=CARTESIAN_POINT('Ctrl Pts',(0.0548532617164176,-0.0595300000000001,
-1.12247250791414));
#21044=CARTESIAN_POINT('',(0.437601487681057,-0.05953,-1.03511272300331));
#21045=CARTESIAN_POINT('Origin',(0.,-0.05953,0.));
#21046=CARTESIAN_POINT('',(0.911784794170997,-0.05953,-0.656964154625313));
#21047=CARTESIAN_POINT('Ctrl Pts',(0.437601487681056,-0.0595300000000001,
-1.03511272300331));
#21048=CARTESIAN_POINT('Ctrl Pts',(0.440685038163619,-0.0762225747374255,
-1.03380912944435));
#21049=CARTESIAN_POINT('Ctrl Pts',(0.445111721969657,-0.0928409665394228,
-1.03192403056628));
#21050=CARTESIAN_POINT('Ctrl Pts',(0.463236132117164,-0.144299303100741,
-1.0239876538093));
#21051=CARTESIAN_POINT('Ctrl Pts',(0.481944444320713,-0.177024326825049,
-1.01550068154148));
#21052=CARTESIAN_POINT('Ctrl Pts',(0.522002043615455,-0.227269801620064,
-0.995447160474328));
#21053=CARTESIAN_POINT('Ctrl Pts',(0.548158511259203,-0.251265615809407,
-0.981446681891443));
#21054=CARTESIAN_POINT('Ctrl Pts',(0.591247219971725,-0.279889827963178,
-0.955972930713954));
#21055=CARTESIAN_POINT('Ctrl Pts',(0.613307674922609,-0.290879136862659,
-0.942092777160053));
#21056=CARTESIAN_POINT('Ctrl Pts',(0.657923009631182,-0.305251990234487,
-0.91149460735272));
#21057=CARTESIAN_POINT('Ctrl Pts',(0.680463863683393,-0.308638795020976,
-0.894757676234429));
#21058=CARTESIAN_POINT('Ctrl Pts',(0.720906778729542,-0.308638795020976,
-0.862505527716294));
#21059=CARTESIAN_POINT('Ctrl Pts',(0.742239891936899,-0.305251990234488,
-0.844254137480381));
#21060=CARTESIAN_POINT('Ctrl Pts',(0.781998747691872,-0.290879136862659,
-0.80756613568454));
#21061=CARTESIAN_POINT('Ctrl Pts',(0.800439809856112,-0.279889827963178,
-0.789147407129765));
#21062=CARTESIAN_POINT('Ctrl Pts',(0.834863020612702,-0.251265615809407,
-0.752807465209441));
#21063=CARTESIAN_POINT('Ctrl Pts',(0.854332839576145,-0.227269801620064,
-0.73042219438957));
#21064=CARTESIAN_POINT('Ctrl Pts',(0.882797231409153,-0.177024326825049,
-0.695831250979106));
#21065=CARTESIAN_POINT('Ctrl Pts',(0.895234408667242,-0.144299303100741,
-0.679480524217551));
#21066=CARTESIAN_POINT('Ctrl Pts',(0.907004864562642,-0.0928409665394228,
-0.663576540841106));
#21067=CARTESIAN_POINT('Ctrl Pts',(0.909827729890942,-0.0762225747374256,
-0.659680317203144));
#21068=CARTESIAN_POINT('Ctrl Pts',(0.911784794170998,-0.0595300000000001,
-0.656964154625312));
#21069=CARTESIAN_POINT('',(1.08212377959455,-0.05953,-0.303251606722892));
#21070=CARTESIAN_POINT('Origin',(0.,-0.05953,0.));
#21071=CARTESIAN_POINT('',(1.08212377959455,-0.05953,0.303251606722892));
#21072=CARTESIAN_POINT('Ctrl Pts',(1.08212377959455,-0.0595300000000001,
-0.303251606722892));
#21073=CARTESIAN_POINT('Ctrl Pts',(1.0830271513892,-0.0762225747374255,
-0.300028012588062));
#21074=CARTESIAN_POINT('Ctrl Pts',(1.08431331394788,-0.0928409665394228,
-0.2953917518996));
#21075=CARTESIAN_POINT('Ctrl Pts',(1.08940878963422,-0.144299303100741,
-0.276273267473431));
#21076=CARTESIAN_POINT('Ctrl Pts',(1.09443784939331,-0.177024326825049,
-0.256354979351213));
#21077=CARTESIAN_POINT('Ctrl Pts',(1.10373487993589,-0.227269801620064,
-0.212533521233765));
#21078=CARTESIAN_POINT('Ctrl Pts',(1.10909715583869,-0.251265615809407,
-0.183354415742157));
#21079=CARTESIAN_POINT('Ctrl Pts',(1.1160463456491,-0.279889827963178,-0.133783682657561));
#21080=CARTESIAN_POINT('Ctrl Pts',(1.11894887330541,-0.290879136862659,
-0.107881990270302));
#21081=CARTESIAN_POINT('Ctrl Pts',(1.12284346704144,-0.305251990234488,
-0.0539226701638766));
#21082=CARTESIAN_POINT('Ctrl Pts',(1.123812,-0.308638795020976,-0.025864214957475));
#21083=CARTESIAN_POINT('Ctrl Pts',(1.123812,-0.308638795020976,0.025864214957475));
#21084=CARTESIAN_POINT('Ctrl Pts',(1.12284346704144,-0.305251990234488,
0.0539226701638766));
#21085=CARTESIAN_POINT('Ctrl Pts',(1.11894887330541,-0.290879136862659,
0.107881990270302));
#21086=CARTESIAN_POINT('Ctrl Pts',(1.1160463456491,-0.279889827963178,0.133783682657561));
#21087=CARTESIAN_POINT('Ctrl Pts',(1.10909715583869,-0.251265615809407,
0.183354415742157));
#21088=CARTESIAN_POINT('Ctrl Pts',(1.10373487993589,-0.227269801620064,
0.212533521233765));
#21089=CARTESIAN_POINT('Ctrl Pts',(1.09443784939331,-0.177024326825049,
0.256354979351213));
#21090=CARTESIAN_POINT('Ctrl Pts',(1.08940878963422,-0.144299303100741,
0.276273267473431));
#21091=CARTESIAN_POINT('Ctrl Pts',(1.08431331394788,-0.0928409665394228,
0.2953917518996));
#21092=CARTESIAN_POINT('Ctrl Pts',(1.0830271513892,-0.0762225747374255,
0.300028012588062));
#21093=CARTESIAN_POINT('Ctrl Pts',(1.08212377959455,-0.0595300000000001,
0.303251606722892));
#21094=CARTESIAN_POINT('Origin',(0.,-0.05953,0.));
#21095=CARTESIAN_POINT('Origin',(0.,-0.05953,0.));
#21096=CARTESIAN_POINT('',(0.0589974094846122,-0.05953,1.07456964270265));
#21097=CARTESIAN_POINT('Origin',(0.,-0.05953,0.));
#21098=CARTESIAN_POINT('Origin',(-0.244773027351946,-0.05953,1.07242070340001));
#21099=CARTESIAN_POINT('Origin',(-0.244773027351946,0.,1.07242070340001));
#21100=CARTESIAN_POINT('',(-0.519393123750572,-0.05953,0.942555777842682));
#21101=CARTESIAN_POINT('Ctrl Pts',(-0.519393123750572,-0.05953,0.942555777842682));
#21102=CARTESIAN_POINT('Ctrl Pts',(-0.513714466572041,-0.0925528133349865,
0.945684988399766));
#21103=CARTESIAN_POINT('Ctrl Pts',(-0.503136848051455,-0.124911173756694,
0.951483858396181));
#21104=CARTESIAN_POINT('Ctrl Pts',(-0.47593627990192,-0.177924977804098,
0.965323333309091));
#21105=CARTESIAN_POINT('Ctrl Pts',(-0.460931856495794,-0.199697230012983,
0.972669835243841));
#21106=CARTESIAN_POINT('Ctrl Pts',(-0.426157505475872,-0.237895043532788,
0.988400002689705));
#21107=CARTESIAN_POINT('Ctrl Pts',(-0.406380688682952,-0.254319232363049,
0.996771768218699));
#21108=CARTESIAN_POINT('Ctrl Pts',(-0.364750145543744,-0.28018331644634,
1.01272583306292));
#21109=CARTESIAN_POINT('Ctrl Pts',(-0.340838910881557,-0.29104845371857,
1.02112815447116));
#21110=CARTESIAN_POINT('Ctrl Pts',(-0.290495481564827,-0.30527573347708,
1.036574285215));
#21111=CARTESIAN_POINT('Ctrl Pts',(-0.264056468041074,-0.308638795020976,
1.04359501395068));
#21112=CARTESIAN_POINT('Ctrl Pts',(-0.214892249704082,-0.308638795020976,
1.05481642595959));
#21113=CARTESIAN_POINT('Ctrl Pts',(-0.188025341585962,-0.30527573347708,
1.05996242598502));
#21114=CARTESIAN_POINT('Ctrl Pts',(-0.135965654106109,-0.29104845371857,
1.06788913840721));
#21115=CARTESIAN_POINT('Ctrl Pts',(-0.110776745452494,-0.28018331644634,
1.07069360430242));
#21116=CARTESIAN_POINT('Ctrl Pts',(-0.0663467128214646,-0.254319232363049,
1.07438230428002));
#21117=CARTESIAN_POINT('Ctrl Pts',(-0.0448960436540983,-0.237895043532788,
1.07542044338697));
#21118=CARTESIAN_POINT('Ctrl Pts',(-0.00674037211528124,-0.199697230012983,
1.07633607767727));
#21119=CARTESIAN_POINT('Ctrl Pts',(0.00996567398334777,-0.177924977804098,
1.07622728347683));
#21120=CARTESIAN_POINT('Ctrl Pts',(0.0404772621979741,-0.124911173756694,
1.07556023164702));
#21121=CARTESIAN_POINT('Ctrl Pts',(0.0525234025782719,-0.0925528133349865,
1.07492508698591));
#21122=CARTESIAN_POINT('Ctrl Pts',(0.0589974094846124,-0.05953,1.07456964270265));
#21123=CARTESIAN_POINT('Origin',(-0.244773027351946,-0.05953,1.07242070340001));
#21124=CARTESIAN_POINT('Origin',(0.,-0.05953,0.));
#21125=CARTESIAN_POINT('',(-0.803348093619616,-0.05953,0.716109245731214));
#21126=CARTESIAN_POINT('Origin',(0.,-0.05953,0.));
#21127=CARTESIAN_POINT('Origin',(-0.991065754692661,-0.05953,0.477272113029314));
#21128=CARTESIAN_POINT('Origin',(-0.991065754692661,0.,0.477272113029314));
#21129=CARTESIAN_POINT('',(-1.06075609691358,-0.05953,0.181596019242328));
#21130=CARTESIAN_POINT('Ctrl Pts',(-1.06075609691358,-0.05953,0.181596019242328));
#21131=CARTESIAN_POINT('Ctrl Pts',(-1.05966202740332,-0.0925528133349865,
0.187986803072856));
#21132=CARTESIAN_POINT('Ctrl Pts',(-1.05760072925372,-0.124911173756694,
0.199872254546857));
#21133=CARTESIAN_POINT('Ctrl Pts',(-1.05146158959546,-0.177924977804098,
0.22976728653846));
#21134=CARTESIAN_POINT('Ctrl Pts',(-1.04785021111757,-0.199697230012983,
0.246078686169301));
#21135=CARTESIAN_POINT('Ctrl Pts',(-1.03846709802406,-0.237895043532788,
0.283073967563097));
#21136=CARTESIAN_POINT('Ctrl Pts',(-1.03268176429485,-0.254319232363049,
0.303755815985685));
#21137=CARTESIAN_POINT('Ctrl Pts',(-1.01919893537026,-0.28018331644634,
0.346251081972725));
#21138=CARTESIAN_POINT('Ctrl Pts',(-1.01085972381132,-0.29104845371857,
0.370184399726282));
#21139=CARTESIAN_POINT('Ctrl Pts',(-0.99154738033959,-0.30527573347708,
0.419174982698463));
#21140=CARTESIAN_POINT('Ctrl Pts',(-0.980551951791748,-0.308638795020976,
0.444223188605045));
#21141=CARTESIAN_POINT('Ctrl Pts',(-0.958671816228589,-0.308638795020976,
0.489657758261848));
#21142=CARTESIAN_POINT('Ctrl Pts',(-0.945943877838127,-0.30527573347708,
0.51387163140139));
#21143=CARTESIAN_POINT('Ctrl Pts',(-0.91968254693063,-0.29104845371857,
0.559515758398093));
#21144=CARTESIAN_POINT('Ctrl Pts',(-0.906170138993533,-0.28018331644634,
0.580957796077825));
#21145=CARTESIAN_POINT('Ctrl Pts',(-0.8813524085237,-0.254319232363049,
0.617994461173994));
#21146=CARTESIAN_POINT('Ctrl Pts',(-0.868789784891799,-0.237895043532788,
0.635412538795143));
#21147=CARTESIAN_POINT('Ctrl Pts',(-0.845715984518854,-0.199697230012983,
0.66581473268113));
#21148=CARTESIAN_POINT('Ctrl Pts',(-0.835214876415962,-0.177924977804098,
0.678808213394124));
#21149=CARTESIAN_POINT('Ctrl Pts',(-0.815669690204649,-0.124911173756694,
0.702247233627224));
#21150=CARTESIAN_POINT('Ctrl Pts',(-0.807662468433796,-0.0925528133349865,
0.711269279199861));
#21151=CARTESIAN_POINT('Ctrl Pts',(-0.803348093619616,-0.05953,0.716109245731214));
#21152=CARTESIAN_POINT('Origin',(-0.991065754692661,-0.05953,0.477272113029314));
#21153=CARTESIAN_POINT('Origin',(0.,-0.05953,0.));
#21154=CARTESIAN_POINT('',(-1.076188,-0.05953,1.31795018948079E-16));
#21155=CARTESIAN_POINT('Origin',(0.,-0.05953,0.));
#21156=CARTESIAN_POINT('',(-1.06075609691358,-0.05953,-0.181596019242328));
#21157=CARTESIAN_POINT('Origin',(0.,-0.05953,0.));
#21158=CARTESIAN_POINT('Origin',(-0.991065754692661,-0.05953,-0.477272113029314));
#21159=CARTESIAN_POINT('Origin',(-0.991065754692661,0.,-0.477272113029314));
#21160=CARTESIAN_POINT('',(-0.803348093619616,-0.05953,-0.716109245731215));
#21161=CARTESIAN_POINT('Ctrl Pts',(-0.803348093619616,-0.05953,-0.716109245731215));
#21162=CARTESIAN_POINT('Ctrl Pts',(-0.807662468433795,-0.0925528133349865,
-0.711269279199862));
#21163=CARTESIAN_POINT('Ctrl Pts',(-0.815669690204649,-0.124911173756694,
-0.702247233627224));
#21164=CARTESIAN_POINT('Ctrl Pts',(-0.835214876415962,-0.177924977804098,
-0.678808213394124));
#21165=CARTESIAN_POINT('Ctrl Pts',(-0.845715984518854,-0.199697230012983,
-0.66581473268113));
#21166=CARTESIAN_POINT('Ctrl Pts',(-0.868789784891799,-0.237895043532788,
-0.635412538795143));
#21167=CARTESIAN_POINT('Ctrl Pts',(-0.8813524085237,-0.254319232363049,
-0.617994461173994));
#21168=CARTESIAN_POINT('Ctrl Pts',(-0.906170138993533,-0.28018331644634,
-0.580957796077826));
#21169=CARTESIAN_POINT('Ctrl Pts',(-0.91968254693063,-0.29104845371857,
-0.559515758398093));
#21170=CARTESIAN_POINT('Ctrl Pts',(-0.945943877838127,-0.30527573347708,
-0.51387163140139));
#21171=CARTESIAN_POINT('Ctrl Pts',(-0.958671816228589,-0.308638795020976,
-0.489657758261848));
#21172=CARTESIAN_POINT('Ctrl Pts',(-0.980551951791748,-0.308638795020976,
-0.444223188605045));
#21173=CARTESIAN_POINT('Ctrl Pts',(-0.99154738033959,-0.30527573347708,
-0.419174982698463));
#21174=CARTESIAN_POINT('Ctrl Pts',(-1.01085972381132,-0.29104845371857,
-0.370184399726282));
#21175=CARTESIAN_POINT('Ctrl Pts',(-1.01919893537026,-0.28018331644634,
-0.346251081972725));
#21176=CARTESIAN_POINT('Ctrl Pts',(-1.03268176429485,-0.254319232363049,
-0.303755815985685));
#21177=CARTESIAN_POINT('Ctrl Pts',(-1.03846709802406,-0.237895043532788,
-0.283073967563097));
#21178=CARTESIAN_POINT('Ctrl Pts',(-1.04785021111757,-0.199697230012983,
-0.246078686169302));
#21179=CARTESIAN_POINT('Ctrl Pts',(-1.05146158959546,-0.177924977804098,
-0.229767286538461));
#21180=CARTESIAN_POINT('Ctrl Pts',(-1.05760072925372,-0.124911173756694,
-0.199872254546858));
#21181=CARTESIAN_POINT('Ctrl Pts',(-1.05966202740332,-0.0925528133349864,
-0.187986803072857));
#21182=CARTESIAN_POINT('Ctrl Pts',(-1.06075609691358,-0.05953,-0.181596019242328));
#21183=CARTESIAN_POINT('Origin',(-0.991065754692661,-0.05953,-0.477272113029314));
#21184=CARTESIAN_POINT('Origin',(0.,-0.05953,0.));
#21185=CARTESIAN_POINT('',(-0.519393123750572,-0.05953,-0.942555777842682));
#21186=CARTESIAN_POINT('Origin',(0.,-0.05953,0.));
#21187=CARTESIAN_POINT('Origin',(-0.244773027351946,-0.05953,-1.07242070340001));
#21188=CARTESIAN_POINT('Origin',(-0.244773027351946,0.,-1.07242070340001));
#21189=CARTESIAN_POINT('',(0.0589974094846125,-0.05953,-1.07456964270265));
#21190=CARTESIAN_POINT('Ctrl Pts',(0.0589974094846127,-0.05953,-1.07456964270265));
#21191=CARTESIAN_POINT('Ctrl Pts',(0.0525234025782722,-0.0925528133349865,
-1.07492508698591));
#21192=CARTESIAN_POINT('Ctrl Pts',(0.0404772621979744,-0.124911173756694,
-1.07556023164702));
#21193=CARTESIAN_POINT('Ctrl Pts',(0.0099656739833481,-0.177924977804098,
-1.07622728347683));
#21194=CARTESIAN_POINT('Ctrl Pts',(-0.00674037211528096,-0.199697230012983,
-1.07633607767727));
#21195=CARTESIAN_POINT('Ctrl Pts',(-0.044896043654098,-0.237895043532788,
-1.07542044338697));
#21196=CARTESIAN_POINT('Ctrl Pts',(-0.0663467128214644,-0.254319232363049,
-1.07438230428002));
#21197=CARTESIAN_POINT('Ctrl Pts',(-0.110776745452493,-0.28018331644634,
-1.07069360430242));
#21198=CARTESIAN_POINT('Ctrl Pts',(-0.135965654106109,-0.29104845371857,
-1.06788913840721));
#21199=CARTESIAN_POINT('Ctrl Pts',(-0.188025341585962,-0.30527573347708,
-1.05996242598502));
#21200=CARTESIAN_POINT('Ctrl Pts',(-0.214892249704082,-0.308638795020976,
-1.05481642595959));
#21201=CARTESIAN_POINT('Ctrl Pts',(-0.264056468041074,-0.308638795020976,
-1.04359501395068));
#21202=CARTESIAN_POINT('Ctrl Pts',(-0.290495481564827,-0.30527573347708,
-1.036574285215));
#21203=CARTESIAN_POINT('Ctrl Pts',(-0.340838910881557,-0.291048453718569,
-1.02112815447116));
#21204=CARTESIAN_POINT('Ctrl Pts',(-0.364750145543744,-0.28018331644634,
-1.01272583306292));
#21205=CARTESIAN_POINT('Ctrl Pts',(-0.406380688682952,-0.254319232363049,
-0.996771768218699));
#21206=CARTESIAN_POINT('Ctrl Pts',(-0.426157505475872,-0.237895043532788,
-0.988400002689705));
#21207=CARTESIAN_POINT('Ctrl Pts',(-0.460931856495794,-0.199697230012983,
-0.972669835243841));
#21208=CARTESIAN_POINT('Ctrl Pts',(-0.475936279901919,-0.177924977804098,
-0.965323333309091));
#21209=CARTESIAN_POINT('Ctrl Pts',(-0.503136848051454,-0.124911173756694,
-0.951483858396181));
#21210=CARTESIAN_POINT('Ctrl Pts',(-0.513714466572041,-0.0925528133349865,
-0.945684988399766));
#21211=CARTESIAN_POINT('Ctrl Pts',(-0.519393123750572,-0.05953,-0.942555777842682));
#21212=CARTESIAN_POINT('Origin',(-0.244773027351946,-0.05953,-1.07242070340001));
#21213=CARTESIAN_POINT('Origin',(0.,-0.05953,0.));
#21214=CARTESIAN_POINT('',(0.413083465285518,-0.05953,-0.993751811093549));
#21215=CARTESIAN_POINT('Origin',(0.,-0.05953,0.));
#21216=CARTESIAN_POINT('Origin',(0.685838782044607,-0.05953,-0.860014630714833));
#21217=CARTESIAN_POINT('Origin',(0.685838782044607,0.,-0.860014630714833));
#21218=CARTESIAN_POINT('',(0.876916659919095,-0.05953,-0.623857181492959));
#21219=CARTESIAN_POINT('Ctrl Pts',(0.876916659919095,-0.05953,-0.623857181492958));
#21220=CARTESIAN_POINT('Ctrl Pts',(0.873158080166742,-0.0925528133349865,
-0.62914037979579));
#21221=CARTESIAN_POINT('Ctrl Pts',(0.866144010579847,-0.124911173756694,
-0.638954437806245));
#21222=CARTESIAN_POINT('Ctrl Pts',(0.847641868610495,-0.177924977804098,
-0.663225258065736));
#21223=CARTESIAN_POINT('Ctrl Pts',(0.837310877969633,-0.199697230012983,
-0.676354402927683));
#21224=CARTESIAN_POINT('Ctrl Pts',(0.81280533416753,-0.237895043532788,
-0.705614819529209));
#21225=CARTESIAN_POINT('Ctrl Pts',(0.798619410861634,-0.254319232363049,
-0.721738358858166));
#21226=CARTESIAN_POINT('Ctrl Pts',(0.768033796848072,-0.28018331644634,
-0.754175290318038));
#21227=CARTESIAN_POINT('Ctrl Pts',(0.750136149454208,-0.29104845371857,
-0.772120216227122));
#21228=CARTESIAN_POINT('Ctrl Pts',(0.711480111898423,-0.30527573347708,
-0.807879894508811));
#21229=CARTESIAN_POINT('Ctrl Pts',(0.690705563850638,-0.308638795020976,
-0.825676810575913));
#21230=CARTESIAN_POINT('Ctrl Pts',(0.651278921914856,-0.308638795020976,
-0.857118508332695));
#21231=CARTESIAN_POINT('Ctrl Pts',(0.629305439856167,-0.30527573347708,
-0.873412008702649));
#21232=CARTESIAN_POINT('Ctrl Pts',(0.585840553788742,-0.29104845371857,
-0.903141581680914));
#21233=CARTESIAN_POINT('Ctrl Pts',(0.564362943424239,-0.28018331644634,
-0.916597376014514));
#21234=CARTESIAN_POINT('Ctrl Pts',(0.525933334162556,-0.254319232363049,
-0.939198248544427));
#21235=CARTESIAN_POINT('Ctrl Pts',(0.507057380724533,-0.237895043532788,
-0.949440676105255));
#21236=CARTESIAN_POINT('Ctrl Pts',(0.473077587363686,-0.199697230012983,
-0.966820759530997));
#21237=CARTESIAN_POINT('Ctrl Pts',(0.457978755888596,-0.177924977804098,
-0.973971221090534));
#21238=CARTESIAN_POINT('Ctrl Pts',(0.430199341854858,-0.124911173756694,
-0.986608710139579));
#21239=CARTESIAN_POINT('Ctrl Pts',(0.419070565453384,-0.0925528133349865,
-0.991263089003441));
#21240=CARTESIAN_POINT('Ctrl Pts',(0.413083465285518,-0.05953,-0.993751811093549));
#21241=CARTESIAN_POINT('Origin',(0.685838782044607,-0.05953,-0.860014630714833));
#21242=CARTESIAN_POINT('Origin',(0.,-0.208355,0.));
#21243=CARTESIAN_POINT('',(-1.076188,-0.35718,1.31795018948079E-16));
#21244=CARTESIAN_POINT('Origin',(0.,-0.35718,0.));
#21245=CARTESIAN_POINT('',(-1.076188,-0.208355,1.31795018948079E-16));
#21246=CARTESIAN_POINT('',(1.03449977959455,-0.05953,0.296632461748266));
#21247=CARTESIAN_POINT('Origin',(0.,-0.05953,0.));
#21248=CARTESIAN_POINT('',(1.03449977959455,-0.05953,-0.296632461748266));
#21249=CARTESIAN_POINT('Ctrl Pts',(1.03449977959455,-0.05953,0.296632461748267));
#21250=CARTESIAN_POINT('Ctrl Pts',(1.03628691421076,-0.0925528133349865,
0.290399865505497));
#21251=CARTESIAN_POINT('Ctrl Pts',(1.03958665287714,-0.124911173756694,
0.278797079997872));
#21252=CARTESIAN_POINT('Ctrl Pts',(1.0470264474309,-0.177924977804098,0.249198913998601));
#21253=CARTESIAN_POINT('Ctrl Pts',(1.05084995891418,-0.199697230012983,
0.232935932341942));
#21254=CARTESIAN_POINT('Ctrl Pts',(1.05844771715377,-0.237895043532788,
0.195533155353269));
#21255=CARTESIAN_POINT('Ctrl Pts',(1.06220882929878,-0.254319232363049,
0.17438929156337));
#21256=CARTESIAN_POINT('Ctrl Pts',(1.06849922508772,-0.28018331644634,0.130252399648131));
#21257=CARTESIAN_POINT('Ctrl Pts',(1.07137013248666,-0.29104845371857,0.105070977154072));
#21258=CARTESIAN_POINT('Ctrl Pts',(1.07522652957392,-0.30527573347708,0.0525526752791107));
#21259=CARTESIAN_POINT('Ctrl Pts',(1.076188,-0.308638795020976,0.025214283908933));
#21260=CARTESIAN_POINT('Ctrl Pts',(1.076188,-0.308638795020976,-0.025214283908933));
#21261=CARTESIAN_POINT('Ctrl Pts',(1.07522652957392,-0.30527573347708,-0.0525526752791107));
#21262=CARTESIAN_POINT('Ctrl Pts',(1.07137013248666,-0.29104845371857,-0.105070977154072));
#21263=CARTESIAN_POINT('Ctrl Pts',(1.06849922508772,-0.28018331644634,-0.130252399648131));
#21264=CARTESIAN_POINT('Ctrl Pts',(1.06220882929878,-0.254319232363049,
-0.17438929156337));
#21265=CARTESIAN_POINT('Ctrl Pts',(1.05844771715377,-0.237895043532788,
-0.195533155353269));
#21266=CARTESIAN_POINT('Ctrl Pts',(1.05084995891418,-0.199697230012983,
-0.232935932341942));
#21267=CARTESIAN_POINT('Ctrl Pts',(1.0470264474309,-0.177924977804098,-0.249198913998601));
#21268=CARTESIAN_POINT('Ctrl Pts',(1.03958665287714,-0.124911173756694,
-0.278797079997872));
#21269=CARTESIAN_POINT('Ctrl Pts',(1.03628691421076,-0.0925528133349865,
-0.290399865505497));
#21270=CARTESIAN_POINT('Ctrl Pts',(1.03449977959455,-0.05953,-0.296632461748267));
#21271=CARTESIAN_POINT('Origin',(0.,-0.05953,0.));
#21272=CARTESIAN_POINT('Origin',(0.,-0.05953,0.));
#21273=CARTESIAN_POINT('Origin',(1.1,-0.05953,0.));
#21274=CARTESIAN_POINT('Origin',(1.1,0.,0.));
#21275=CARTESIAN_POINT('Origin',(1.1,-0.05953,0.));
#21276=CARTESIAN_POINT('Origin',(0.,-0.35718,0.));
#21277=CARTESIAN_POINT('Origin',(0.,-0.05953,0.));
#34769=UNCERTAINTY_MEASURE_WITH_UNIT(LENGTH_MEASURE(0.001),#34852,
'DISTANCE_ACCURACY_VALUE',
'Maximum model space distance between geometric entities at asserted c
onnectivities');
#34797=UNCERTAINTY_MEASURE_WITH_UNIT(LENGTH_MEASURE(0.001),#34852,
'DISTANCE_ACCURACY_VALUE',
'Maximum model space distance between geometric entities at asserted c
onnectivities');
#34823=(
GEOMETRIC_REPRESENTATION_CONTEXT(3)
GLOBAL_UNCERTAINTY_ASSIGNED_CONTEXT((#34769))
GLOBAL_UNIT_ASSIGNED_CONTEXT((#34852,#34854,#34855))
REPRESENTATION_CONTEXT('','3D')
);
#34851=(
GEOMETRIC_REPRESENTATION_CONTEXT(3)
GLOBAL_UNCERTAINTY_ASSIGNED_CONTEXT((#34797))
GLOBAL_UNIT_ASSIGNED_CONTEXT((#34852,#34854,#34855))
REPRESENTATION_CONTEXT('','3D')
);
#34852=(
LENGTH_UNIT()
NAMED_UNIT(*)
SI_UNIT(.CENTI.,.METRE.)
);
#34854=(
NAMED_UNIT(*)
PLANE_ANGLE_UNIT()
SI_UNIT($,.RADIAN.)
);
#34855=(
NAMED_UNIT(*)
SI_UNIT($,.STERADIAN.)
SOLID_ANGLE_UNIT()
);
#34881=SHAPE_DEFINITION_REPRESENTATION(#34934,#35098);
#34934=PRODUCT_DEFINITION_SHAPE('',$,#35152);
#35098=SHAPE_REPRESENTATION('',(#14834),#34823);
#35126=PRODUCT_DEFINITION_CONTEXT('part definition',#35287,'design');
#35152=PRODUCT_DEFINITION('Cage','Cage',#35205,#35126);
#35205=PRODUCT_DEFINITION_FORMATION('',$,#35314);
#35287=APPLICATION_CONTEXT(
'Core Data for Automotive Mechanical Design Process');
#35288=PRODUCT_CONTEXT('part definition',#35287,'mechanical');
#35314=PRODUCT('Cage','Cage','Cage',(#35288));
#35405=COLOUR_RGB('Grey',0.48,0.52,0.57);
#35406=FILL_AREA_STYLE_COLOUR('',#35405);
#35407=FILL_AREA_STYLE('',(#35406));
#35408=SURFACE_STYLE_FILL_AREA(#35407);
#35409=SURFACE_SIDE_STYLE('',(#35408));
#35410=SURFACE_STYLE_USAGE(.BOTH.,#35409);
#35411=PRESENTATION_STYLE_ASSIGNMENT((#35410));
ENDSEC;
END-ISO-10303-21;
